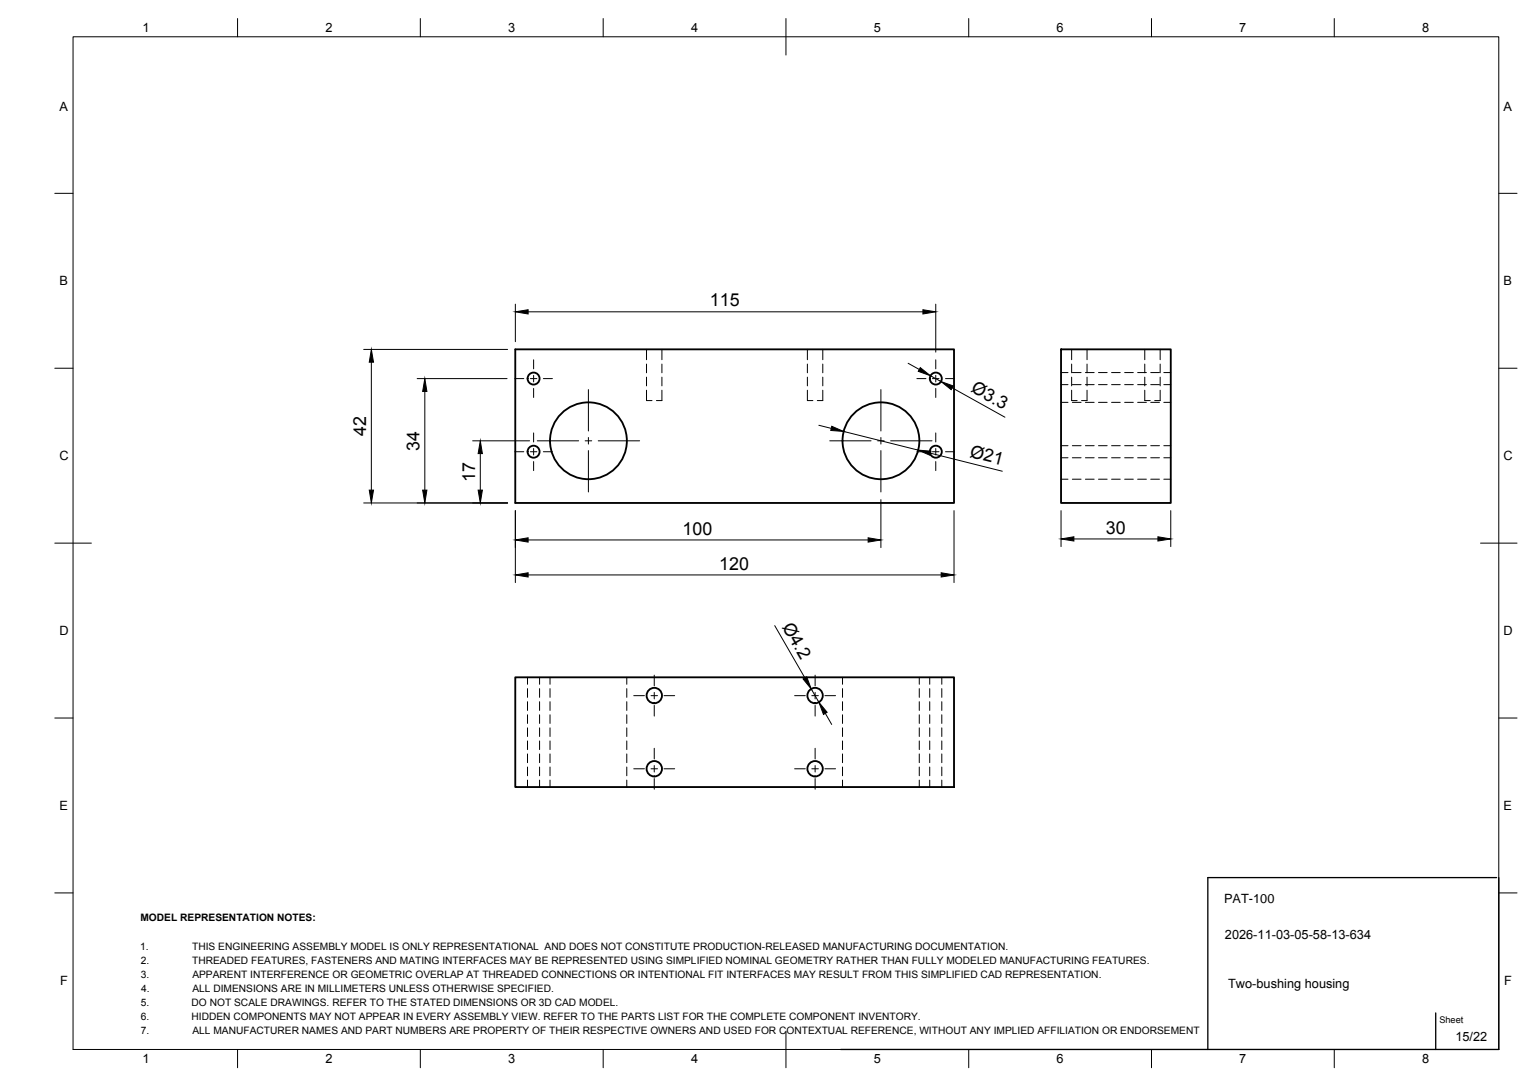
ISO-10303-21;
HEADER;
/* Generated by software containing ST-Developer
 * from STEP Tools, Inc. (www.steptools.com) 
 */

FILE_DESCRIPTION(
/* description */ (''),
/* implementation_level */ '2;1');

FILE_NAME(
/* name */ 'Two-bushing housing.step',
/* time_stamp */ '2026-10-29T16:43:51-07:00',
/* author */ (''),
/* organization */ (''),
/* preprocessor_version */ 'ST-DEVELOPER v20.2',
/* originating_system */ 'Autodesk Translation Framework v15.17.0.0',
/* authorisation */ '');

FILE_SCHEMA (('AUTOMOTIVE_DESIGN { 1 0 10303 214 3 1 1 }'));
ENDSEC;

DATA;
#10=MECHANICAL_DESIGN_GEOMETRIC_PRESENTATION_REPRESENTATION('',(#378),#10292);
#332=SHAPE_REPRESENTATION_RELATIONSHIP('SRR','None',#10429,#355);
#355=ADVANCED_BREP_SHAPE_REPRESENTATION('',(#399),#10281);
#378=STYLED_ITEM('',(#10607),#399);
#399=MANIFOLD_SOLID_BREP('Body1',#5022);
#475=FACE_BOUND('',#1244,.T.);
#476=FACE_BOUND('',#1245,.T.);
#477=FACE_BOUND('',#1246,.T.);
#478=FACE_BOUND('',#1247,.T.);
#479=FACE_BOUND('',#1248,.T.);
#480=FACE_BOUND('',#1249,.T.);
#481=FACE_BOUND('',#1252,.T.);
#482=FACE_BOUND('',#1253,.T.);
#483=FACE_BOUND('',#1254,.T.);
#484=FACE_BOUND('',#1255,.T.);
#485=FACE_BOUND('',#1256,.T.);
#486=FACE_BOUND('',#1257,.T.);
#487=FACE_BOUND('',#1259,.T.);
#488=FACE_BOUND('',#1260,.T.);
#489=FACE_BOUND('',#1261,.T.);
#490=FACE_BOUND('',#1262,.T.);
#634=PLANE('',#5584);
#635=PLANE('',#5588);
#636=PLANE('',#5592);
#637=PLANE('',#5596);
#638=PLANE('',#5603);
#639=PLANE('',#5604);
#640=PLANE('',#5605);
#641=PLANE('',#5606);
#642=PLANE('',#5607);
#643=PLANE('',#5608);
#871=FACE_OUTER_BOUND('',#1228,.T.);
#872=FACE_OUTER_BOUND('',#1229,.T.);
#873=FACE_OUTER_BOUND('',#1230,.T.);
#874=FACE_OUTER_BOUND('',#1231,.T.);
#875=FACE_OUTER_BOUND('',#1232,.T.);
#876=FACE_OUTER_BOUND('',#1233,.T.);
#877=FACE_OUTER_BOUND('',#1234,.T.);
#878=FACE_OUTER_BOUND('',#1235,.T.);
#879=FACE_OUTER_BOUND('',#1236,.T.);
#880=FACE_OUTER_BOUND('',#1237,.T.);
#881=FACE_OUTER_BOUND('',#1238,.T.);
#882=FACE_OUTER_BOUND('',#1239,.T.);
#883=FACE_OUTER_BOUND('',#1240,.T.);
#884=FACE_OUTER_BOUND('',#1241,.T.);
#885=FACE_OUTER_BOUND('',#1242,.T.);
#886=FACE_OUTER_BOUND('',#1243,.T.);
#887=FACE_OUTER_BOUND('',#1250,.T.);
#888=FACE_OUTER_BOUND('',#1251,.T.);
#889=FACE_OUTER_BOUND('',#1258,.T.);
#890=FACE_OUTER_BOUND('',#1263,.T.);
#1228=EDGE_LOOP('',(#4127,#4128,#4129,#4130));
#1229=EDGE_LOOP('',(#4131,#4132,#4133,#4134));
#1230=EDGE_LOOP('',(#4135,#4136,#4137,#4138));
#1231=EDGE_LOOP('',(#4139,#4140,#4141,#4142));
#1232=EDGE_LOOP('',(#4143,#4144,#4145,#4146));
#1233=EDGE_LOOP('',(#4147));
#1234=EDGE_LOOP('',(#4148,#4149,#4150,#4151));
#1235=EDGE_LOOP('',(#4152));
#1236=EDGE_LOOP('',(#4153,#4154,#4155,#4156));
#1237=EDGE_LOOP('',(#4157));
#1238=EDGE_LOOP('',(#4158,#4159,#4160,#4161));
#1239=EDGE_LOOP('',(#4162));
#1240=EDGE_LOOP('',(#4163,#4164,#4165,#4166));
#1241=EDGE_LOOP('',(#4167,#4168,#4169,#4170));
#1242=EDGE_LOOP('',(#4171,#4172,#4173,#4174));
#1243=EDGE_LOOP('',(#4175,#4176,#4177,#4178));
#1244=EDGE_LOOP('',(#4179));
#1245=EDGE_LOOP('',(#4180));
#1246=EDGE_LOOP('',(#4181));
#1247=EDGE_LOOP('',(#4182));
#1248=EDGE_LOOP('',(#4183));
#1249=EDGE_LOOP('',(#4184));
#1250=EDGE_LOOP('',(#4185,#4186,#4187,#4188));
#1251=EDGE_LOOP('',(#4189,#4190,#4191,#4192));
#1252=EDGE_LOOP('',(#4193));
#1253=EDGE_LOOP('',(#4194));
#1254=EDGE_LOOP('',(#4195));
#1255=EDGE_LOOP('',(#4196));
#1256=EDGE_LOOP('',(#4197));
#1257=EDGE_LOOP('',(#4198));
#1258=EDGE_LOOP('',(#4199,#4200,#4201,#4202));
#1259=EDGE_LOOP('',(#4203));
#1260=EDGE_LOOP('',(#4204));
#1261=EDGE_LOOP('',(#4205));
#1262=EDGE_LOOP('',(#4206));
#1263=EDGE_LOOP('',(#4207,#4208,#4209,#4210));
#1644=LINE('',#9621,#2036);
#1645=LINE('',#9627,#2037);
#1646=LINE('',#9633,#2038);
#1647=LINE('',#9639,#2039);
#1648=LINE('',#9645,#2040);
#1649=LINE('',#9652,#2041);
#1650=LINE('',#9659,#2042);
#1651=LINE('',#9666,#2043);
#1652=LINE('',#9673,#2044);
#1653=LINE('',#9679,#2045);
#1654=LINE('',#9684,#2046);
#1655=LINE('',#9686,#2047);
#1656=LINE('',#9688,#2048);
#1657=LINE('',#9689,#2049);
#1658=LINE('',#9692,#2050);
#1659=LINE('',#9694,#2051);
#1660=LINE('',#9695,#2052);
#1661=LINE('',#9698,#2053);
#1662=LINE('',#9700,#2054);
#1663=LINE('',#9701,#2055);
#1664=LINE('',#9703,#2056);
#1665=LINE('',#9704,#2057);
#2036=VECTOR('',#6661,0.165);
#2037=VECTOR('',#6668,0.165);
#2038=VECTOR('',#6675,0.165);
#2039=VECTOR('',#6682,0.165);
#2040=VECTOR('',#6689,0.210000000000001);
#2041=VECTOR('',#6698,0.210000000000001);
#2042=VECTOR('',#6707,0.210000000000001);
#2043=VECTOR('',#6716,0.210000000000001);
#2044=VECTOR('',#6725,1.05);
#2045=VECTOR('',#6732,1.05);
#2046=VECTOR('',#6737,1.);
#2047=VECTOR('',#6738,1.);
#2048=VECTOR('',#6739,1.);
#2049=VECTOR('',#6740,1.);
#2050=VECTOR('',#6743,1.);
#2051=VECTOR('',#6744,1.);
#2052=VECTOR('',#6745,1.);
#2053=VECTOR('',#6748,1.);
#2054=VECTOR('',#6749,1.);
#2055=VECTOR('',#6750,1.);
#2056=VECTOR('',#6753,1.);
#2057=VECTOR('',#6754,1.);
#2298=CIRCLE('',#5570,0.165);
#2299=CIRCLE('',#5571,0.165);
#2300=CIRCLE('',#5573,0.165);
#2301=CIRCLE('',#5574,0.165);
#2302=CIRCLE('',#5576,0.165);
#2303=CIRCLE('',#5577,0.165);
#2304=CIRCLE('',#5579,0.165);
#2305=CIRCLE('',#5580,0.165);
#2306=CIRCLE('',#5582,0.210000000000001);
#2307=CIRCLE('',#5583,0.210000000000001);
#2308=CIRCLE('',#5586,0.210000000000001);
#2309=CIRCLE('',#5587,0.210000000000001);
#2310=CIRCLE('',#5590,0.210000000000001);
#2311=CIRCLE('',#5591,0.210000000000001);
#2312=CIRCLE('',#5594,0.210000000000001);
#2313=CIRCLE('',#5595,0.210000000000001);
#2314=CIRCLE('',#5598,1.05);
#2315=CIRCLE('',#5599,1.05);
#2316=CIRCLE('',#5601,1.05);
#2317=CIRCLE('',#5602,1.05);
#2629=VERTEX_POINT('',#9618);
#2630=VERTEX_POINT('',#9620);
#2631=VERTEX_POINT('',#9624);
#2632=VERTEX_POINT('',#9626);
#2633=VERTEX_POINT('',#9630);
#2634=VERTEX_POINT('',#9632);
#2635=VERTEX_POINT('',#9636);
#2636=VERTEX_POINT('',#9638);
#2637=VERTEX_POINT('',#9642);
#2638=VERTEX_POINT('',#9644);
#2639=VERTEX_POINT('',#9649);
#2640=VERTEX_POINT('',#9651);
#2641=VERTEX_POINT('',#9656);
#2642=VERTEX_POINT('',#9658);
#2643=VERTEX_POINT('',#9663);
#2644=VERTEX_POINT('',#9665);
#2645=VERTEX_POINT('',#9670);
#2646=VERTEX_POINT('',#9672);
#2647=VERTEX_POINT('',#9676);
#2648=VERTEX_POINT('',#9678);
#2649=VERTEX_POINT('',#9682);
#2650=VERTEX_POINT('',#9683);
#2651=VERTEX_POINT('',#9685);
#2652=VERTEX_POINT('',#9687);
#2653=VERTEX_POINT('',#9691);
#2654=VERTEX_POINT('',#9693);
#2655=VERTEX_POINT('',#9697);
#2656=VERTEX_POINT('',#9699);
#3154=EDGE_CURVE('',#2629,#2629,#2298,.T.);
#3155=EDGE_CURVE('',#2629,#2630,#1644,.T.);
#3156=EDGE_CURVE('',#2630,#2630,#2299,.T.);
#3157=EDGE_CURVE('',#2631,#2631,#2300,.T.);
#3158=EDGE_CURVE('',#2631,#2632,#1645,.T.);
#3159=EDGE_CURVE('',#2632,#2632,#2301,.T.);
#3160=EDGE_CURVE('',#2633,#2633,#2302,.T.);
#3161=EDGE_CURVE('',#2633,#2634,#1646,.T.);
#3162=EDGE_CURVE('',#2634,#2634,#2303,.T.);
#3163=EDGE_CURVE('',#2635,#2635,#2304,.T.);
#3164=EDGE_CURVE('',#2635,#2636,#1647,.T.);
#3165=EDGE_CURVE('',#2636,#2636,#2305,.T.);
#3166=EDGE_CURVE('',#2637,#2637,#2306,.T.);
#3167=EDGE_CURVE('',#2637,#2638,#1648,.T.);
#3168=EDGE_CURVE('',#2638,#2638,#2307,.T.);
#3169=EDGE_CURVE('',#2639,#2639,#2308,.T.);
#3170=EDGE_CURVE('',#2639,#2640,#1649,.T.);
#3171=EDGE_CURVE('',#2640,#2640,#2309,.T.);
#3172=EDGE_CURVE('',#2641,#2641,#2310,.T.);
#3173=EDGE_CURVE('',#2641,#2642,#1650,.T.);
#3174=EDGE_CURVE('',#2642,#2642,#2311,.T.);
#3175=EDGE_CURVE('',#2643,#2643,#2312,.T.);
#3176=EDGE_CURVE('',#2643,#2644,#1651,.T.);
#3177=EDGE_CURVE('',#2644,#2644,#2313,.T.);
#3178=EDGE_CURVE('',#2645,#2645,#2314,.T.);
#3179=EDGE_CURVE('',#2645,#2646,#1652,.T.);
#3180=EDGE_CURVE('',#2646,#2646,#2315,.T.);
#3181=EDGE_CURVE('',#2647,#2647,#2316,.T.);
#3182=EDGE_CURVE('',#2647,#2648,#1653,.T.);
#3183=EDGE_CURVE('',#2648,#2648,#2317,.T.);
#3184=EDGE_CURVE('',#2649,#2650,#1654,.T.);
#3185=EDGE_CURVE('',#2650,#2651,#1655,.T.);
#3186=EDGE_CURVE('',#2652,#2651,#1656,.T.);
#3187=EDGE_CURVE('',#2649,#2652,#1657,.T.);
#3188=EDGE_CURVE('',#2653,#2649,#1658,.T.);
#3189=EDGE_CURVE('',#2654,#2652,#1659,.T.);
#3190=EDGE_CURVE('',#2653,#2654,#1660,.T.);
#3191=EDGE_CURVE('',#2655,#2653,#1661,.T.);
#3192=EDGE_CURVE('',#2656,#2654,#1662,.T.);
#3193=EDGE_CURVE('',#2655,#2656,#1663,.T.);
#3194=EDGE_CURVE('',#2650,#2655,#1664,.T.);
#3195=EDGE_CURVE('',#2651,#2656,#1665,.T.);
#4127=ORIENTED_EDGE('',*,*,#3154,.F.);
#4128=ORIENTED_EDGE('',*,*,#3155,.T.);
#4129=ORIENTED_EDGE('',*,*,#3156,.F.);
#4130=ORIENTED_EDGE('',*,*,#3155,.F.);
#4131=ORIENTED_EDGE('',*,*,#3157,.F.);
#4132=ORIENTED_EDGE('',*,*,#3158,.T.);
#4133=ORIENTED_EDGE('',*,*,#3159,.F.);
#4134=ORIENTED_EDGE('',*,*,#3158,.F.);
#4135=ORIENTED_EDGE('',*,*,#3160,.F.);
#4136=ORIENTED_EDGE('',*,*,#3161,.T.);
#4137=ORIENTED_EDGE('',*,*,#3162,.F.);
#4138=ORIENTED_EDGE('',*,*,#3161,.F.);
#4139=ORIENTED_EDGE('',*,*,#3163,.F.);
#4140=ORIENTED_EDGE('',*,*,#3164,.T.);
#4141=ORIENTED_EDGE('',*,*,#3165,.F.);
#4142=ORIENTED_EDGE('',*,*,#3164,.F.);
#4143=ORIENTED_EDGE('',*,*,#3166,.F.);
#4144=ORIENTED_EDGE('',*,*,#3167,.T.);
#4145=ORIENTED_EDGE('',*,*,#3168,.F.);
#4146=ORIENTED_EDGE('',*,*,#3167,.F.);
#4147=ORIENTED_EDGE('',*,*,#3166,.T.);
#4148=ORIENTED_EDGE('',*,*,#3169,.F.);
#4149=ORIENTED_EDGE('',*,*,#3170,.T.);
#4150=ORIENTED_EDGE('',*,*,#3171,.F.);
#4151=ORIENTED_EDGE('',*,*,#3170,.F.);
#4152=ORIENTED_EDGE('',*,*,#3169,.T.);
#4153=ORIENTED_EDGE('',*,*,#3172,.F.);
#4154=ORIENTED_EDGE('',*,*,#3173,.T.);
#4155=ORIENTED_EDGE('',*,*,#3174,.F.);
#4156=ORIENTED_EDGE('',*,*,#3173,.F.);
#4157=ORIENTED_EDGE('',*,*,#3172,.T.);
#4158=ORIENTED_EDGE('',*,*,#3175,.F.);
#4159=ORIENTED_EDGE('',*,*,#3176,.T.);
#4160=ORIENTED_EDGE('',*,*,#3177,.F.);
#4161=ORIENTED_EDGE('',*,*,#3176,.F.);
#4162=ORIENTED_EDGE('',*,*,#3175,.T.);
#4163=ORIENTED_EDGE('',*,*,#3178,.F.);
#4164=ORIENTED_EDGE('',*,*,#3179,.T.);
#4165=ORIENTED_EDGE('',*,*,#3180,.F.);
#4166=ORIENTED_EDGE('',*,*,#3179,.F.);
#4167=ORIENTED_EDGE('',*,*,#3181,.F.);
#4168=ORIENTED_EDGE('',*,*,#3182,.T.);
#4169=ORIENTED_EDGE('',*,*,#3183,.F.);
#4170=ORIENTED_EDGE('',*,*,#3182,.F.);
#4171=ORIENTED_EDGE('',*,*,#3184,.T.);
#4172=ORIENTED_EDGE('',*,*,#3185,.T.);
#4173=ORIENTED_EDGE('',*,*,#3186,.F.);
#4174=ORIENTED_EDGE('',*,*,#3187,.F.);
#4175=ORIENTED_EDGE('',*,*,#3188,.T.);
#4176=ORIENTED_EDGE('',*,*,#3187,.T.);
#4177=ORIENTED_EDGE('',*,*,#3189,.F.);
#4178=ORIENTED_EDGE('',*,*,#3190,.F.);
#4179=ORIENTED_EDGE('',*,*,#3183,.T.);
#4180=ORIENTED_EDGE('',*,*,#3180,.T.);
#4181=ORIENTED_EDGE('',*,*,#3165,.T.);
#4182=ORIENTED_EDGE('',*,*,#3162,.T.);
#4183=ORIENTED_EDGE('',*,*,#3159,.T.);
#4184=ORIENTED_EDGE('',*,*,#3156,.T.);
#4185=ORIENTED_EDGE('',*,*,#3191,.T.);
#4186=ORIENTED_EDGE('',*,*,#3190,.T.);
#4187=ORIENTED_EDGE('',*,*,#3192,.F.);
#4188=ORIENTED_EDGE('',*,*,#3193,.F.);
#4189=ORIENTED_EDGE('',*,*,#3194,.T.);
#4190=ORIENTED_EDGE('',*,*,#3193,.T.);
#4191=ORIENTED_EDGE('',*,*,#3195,.F.);
#4192=ORIENTED_EDGE('',*,*,#3185,.F.);
#4193=ORIENTED_EDGE('',*,*,#3181,.T.);
#4194=ORIENTED_EDGE('',*,*,#3178,.T.);
#4195=ORIENTED_EDGE('',*,*,#3163,.T.);
#4196=ORIENTED_EDGE('',*,*,#3160,.T.);
#4197=ORIENTED_EDGE('',*,*,#3157,.T.);
#4198=ORIENTED_EDGE('',*,*,#3154,.T.);
#4199=ORIENTED_EDGE('',*,*,#3195,.T.);
#4200=ORIENTED_EDGE('',*,*,#3192,.T.);
#4201=ORIENTED_EDGE('',*,*,#3189,.T.);
#4202=ORIENTED_EDGE('',*,*,#3186,.T.);
#4203=ORIENTED_EDGE('',*,*,#3168,.T.);
#4204=ORIENTED_EDGE('',*,*,#3171,.T.);
#4205=ORIENTED_EDGE('',*,*,#3174,.T.);
#4206=ORIENTED_EDGE('',*,*,#3177,.T.);
#4207=ORIENTED_EDGE('',*,*,#3194,.F.);
#4208=ORIENTED_EDGE('',*,*,#3184,.F.);
#4209=ORIENTED_EDGE('',*,*,#3188,.F.);
#4210=ORIENTED_EDGE('',*,*,#3191,.F.);
#4680=CYLINDRICAL_SURFACE('',#5569,0.165);
#4681=CYLINDRICAL_SURFACE('',#5572,0.165);
#4682=CYLINDRICAL_SURFACE('',#5575,0.165);
#4683=CYLINDRICAL_SURFACE('',#5578,0.165);
#4684=CYLINDRICAL_SURFACE('',#5581,0.210000000000001);
#4685=CYLINDRICAL_SURFACE('',#5585,0.210000000000001);
#4686=CYLINDRICAL_SURFACE('',#5589,0.210000000000001);
#4687=CYLINDRICAL_SURFACE('',#5593,0.210000000000001);
#4688=CYLINDRICAL_SURFACE('',#5597,1.05);
#4689=CYLINDRICAL_SURFACE('',#5600,1.05);
#4880=ADVANCED_FACE('',(#871),#4680,.F.);
#4881=ADVANCED_FACE('',(#872),#4681,.F.);
#4882=ADVANCED_FACE('',(#873),#4682,.F.);
#4883=ADVANCED_FACE('',(#874),#4683,.F.);
#4884=ADVANCED_FACE('',(#875),#4684,.F.);
#4885=ADVANCED_FACE('',(#876),#634,.T.);
#4886=ADVANCED_FACE('',(#877),#4685,.F.);
#4887=ADVANCED_FACE('',(#878),#635,.T.);
#4888=ADVANCED_FACE('',(#879),#4686,.F.);
#4889=ADVANCED_FACE('',(#880),#636,.T.);
#4890=ADVANCED_FACE('',(#881),#4687,.F.);
#4891=ADVANCED_FACE('',(#882),#637,.T.);
#4892=ADVANCED_FACE('',(#883),#4688,.F.);
#4893=ADVANCED_FACE('',(#884),#4689,.F.);
#4894=ADVANCED_FACE('',(#885),#638,.T.);
#4895=ADVANCED_FACE('',(#886,#475,#476,#477,#478,#479,#480),#639,.T.);
#4896=ADVANCED_FACE('',(#887),#640,.T.);
#4897=ADVANCED_FACE('',(#888,#481,#482,#483,#484,#485,#486),#641,.T.);
#4898=ADVANCED_FACE('',(#889,#487,#488,#489,#490),#642,.T.);
#4899=ADVANCED_FACE('',(#890),#643,.F.);
#5022=CLOSED_SHELL('',(#4880,#4881,#4882,#4883,#4884,#4885,#4886,#4887,
#4888,#4889,#4890,#4891,#4892,#4893,#4894,#4895,#4896,#4897,#4898,#4899));
#5568=AXIS2_PLACEMENT_3D('',#9616,#6655,#6656);
#5569=AXIS2_PLACEMENT_3D('',#9617,#6657,#6658);
#5570=AXIS2_PLACEMENT_3D('',#9619,#6659,#6660);
#5571=AXIS2_PLACEMENT_3D('',#9622,#6662,#6663);
#5572=AXIS2_PLACEMENT_3D('',#9623,#6664,#6665);
#5573=AXIS2_PLACEMENT_3D('',#9625,#6666,#6667);
#5574=AXIS2_PLACEMENT_3D('',#9628,#6669,#6670);
#5575=AXIS2_PLACEMENT_3D('',#9629,#6671,#6672);
#5576=AXIS2_PLACEMENT_3D('',#9631,#6673,#6674);
#5577=AXIS2_PLACEMENT_3D('',#9634,#6676,#6677);
#5578=AXIS2_PLACEMENT_3D('',#9635,#6678,#6679);
#5579=AXIS2_PLACEMENT_3D('',#9637,#6680,#6681);
#5580=AXIS2_PLACEMENT_3D('',#9640,#6683,#6684);
#5581=AXIS2_PLACEMENT_3D('',#9641,#6685,#6686);
#5582=AXIS2_PLACEMENT_3D('',#9643,#6687,#6688);
#5583=AXIS2_PLACEMENT_3D('',#9646,#6690,#6691);
#5584=AXIS2_PLACEMENT_3D('',#9647,#6692,#6693);
#5585=AXIS2_PLACEMENT_3D('',#9648,#6694,#6695);
#5586=AXIS2_PLACEMENT_3D('',#9650,#6696,#6697);
#5587=AXIS2_PLACEMENT_3D('',#9653,#6699,#6700);
#5588=AXIS2_PLACEMENT_3D('',#9654,#6701,#6702);
#5589=AXIS2_PLACEMENT_3D('',#9655,#6703,#6704);
#5590=AXIS2_PLACEMENT_3D('',#9657,#6705,#6706);
#5591=AXIS2_PLACEMENT_3D('',#9660,#6708,#6709);
#5592=AXIS2_PLACEMENT_3D('',#9661,#6710,#6711);
#5593=AXIS2_PLACEMENT_3D('',#9662,#6712,#6713);
#5594=AXIS2_PLACEMENT_3D('',#9664,#6714,#6715);
#5595=AXIS2_PLACEMENT_3D('',#9667,#6717,#6718);
#5596=AXIS2_PLACEMENT_3D('',#9668,#6719,#6720);
#5597=AXIS2_PLACEMENT_3D('',#9669,#6721,#6722);
#5598=AXIS2_PLACEMENT_3D('',#9671,#6723,#6724);
#5599=AXIS2_PLACEMENT_3D('',#9674,#6726,#6727);
#5600=AXIS2_PLACEMENT_3D('',#9675,#6728,#6729);
#5601=AXIS2_PLACEMENT_3D('',#9677,#6730,#6731);
#5602=AXIS2_PLACEMENT_3D('',#9680,#6733,#6734);
#5603=AXIS2_PLACEMENT_3D('',#9681,#6735,#6736);
#5604=AXIS2_PLACEMENT_3D('',#9690,#6741,#6742);
#5605=AXIS2_PLACEMENT_3D('',#9696,#6746,#6747);
#5606=AXIS2_PLACEMENT_3D('',#9702,#6751,#6752);
#5607=AXIS2_PLACEMENT_3D('',#9705,#6755,#6756);
#5608=AXIS2_PLACEMENT_3D('',#9706,#6757,#6758);
#6655=DIRECTION('axis',(0.,0.,1.));
#6656=DIRECTION('refdir',(1.,0.,0.));
#6657=DIRECTION('center_axis',(1.,0.,0.));
#6658=DIRECTION('ref_axis',(0.,0.,-1.));
#6659=DIRECTION('center_axis',(1.,0.,0.));
#6660=DIRECTION('ref_axis',(0.,0.,-1.));
#6661=DIRECTION('',(1.,0.,0.));
#6662=DIRECTION('center_axis',(-1.,0.,0.));
#6663=DIRECTION('ref_axis',(0.,0.,-1.));
#6664=DIRECTION('center_axis',(1.,0.,0.));
#6665=DIRECTION('ref_axis',(0.,0.,-1.));
#6666=DIRECTION('center_axis',(1.,0.,0.));
#6667=DIRECTION('ref_axis',(0.,0.,-1.));
#6668=DIRECTION('',(1.,0.,0.));
#6669=DIRECTION('center_axis',(-1.,0.,0.));
#6670=DIRECTION('ref_axis',(0.,0.,-1.));
#6671=DIRECTION('center_axis',(1.,0.,0.));
#6672=DIRECTION('ref_axis',(0.,0.,-1.));
#6673=DIRECTION('center_axis',(1.,0.,0.));
#6674=DIRECTION('ref_axis',(0.,0.,-1.));
#6675=DIRECTION('',(1.,0.,0.));
#6676=DIRECTION('center_axis',(-1.,0.,0.));
#6677=DIRECTION('ref_axis',(0.,0.,-1.));
#6678=DIRECTION('center_axis',(1.,0.,0.));
#6679=DIRECTION('ref_axis',(0.,0.,-1.));
#6680=DIRECTION('center_axis',(1.,0.,0.));
#6681=DIRECTION('ref_axis',(0.,0.,-1.));
#6682=DIRECTION('',(1.,0.,0.));
#6683=DIRECTION('center_axis',(-1.,0.,0.));
#6684=DIRECTION('ref_axis',(0.,0.,-1.));
#6685=DIRECTION('center_axis',(0.,0.,1.));
#6686=DIRECTION('ref_axis',(1.,0.,0.));
#6687=DIRECTION('center_axis',(0.,0.,1.));
#6688=DIRECTION('ref_axis',(1.,0.,0.));
#6689=DIRECTION('',(0.,0.,1.));
#6690=DIRECTION('center_axis',(0.,0.,-1.));
#6691=DIRECTION('ref_axis',(1.,0.,0.));
#6692=DIRECTION('center_axis',(0.,0.,1.));
#6693=DIRECTION('ref_axis',(1.,0.,0.));
#6694=DIRECTION('center_axis',(0.,0.,1.));
#6695=DIRECTION('ref_axis',(1.,0.,0.));
#6696=DIRECTION('center_axis',(0.,0.,1.));
#6697=DIRECTION('ref_axis',(1.,0.,0.));
#6698=DIRECTION('',(0.,0.,1.));
#6699=DIRECTION('center_axis',(0.,0.,-1.));
#6700=DIRECTION('ref_axis',(1.,0.,0.));
#6701=DIRECTION('center_axis',(0.,0.,1.));
#6702=DIRECTION('ref_axis',(1.,0.,0.));
#6703=DIRECTION('center_axis',(0.,0.,1.));
#6704=DIRECTION('ref_axis',(1.,0.,0.));
#6705=DIRECTION('center_axis',(0.,0.,1.));
#6706=DIRECTION('ref_axis',(1.,0.,0.));
#6707=DIRECTION('',(0.,0.,1.));
#6708=DIRECTION('center_axis',(0.,0.,-1.));
#6709=DIRECTION('ref_axis',(1.,0.,0.));
#6710=DIRECTION('center_axis',(0.,0.,1.));
#6711=DIRECTION('ref_axis',(1.,0.,0.));
#6712=DIRECTION('center_axis',(0.,0.,1.));
#6713=DIRECTION('ref_axis',(1.,0.,0.));
#6714=DIRECTION('center_axis',(0.,0.,1.));
#6715=DIRECTION('ref_axis',(1.,0.,0.));
#6716=DIRECTION('',(0.,0.,1.));
#6717=DIRECTION('center_axis',(0.,0.,-1.));
#6718=DIRECTION('ref_axis',(1.,0.,0.));
#6719=DIRECTION('center_axis',(0.,0.,1.));
#6720=DIRECTION('ref_axis',(1.,0.,0.));
#6721=DIRECTION('center_axis',(1.,0.,0.));
#6722=DIRECTION('ref_axis',(0.,0.,-1.));
#6723=DIRECTION('center_axis',(1.,0.,0.));
#6724=DIRECTION('ref_axis',(0.,0.,-1.));
#6725=DIRECTION('',(1.,0.,0.));
#6726=DIRECTION('center_axis',(-1.,0.,0.));
#6727=DIRECTION('ref_axis',(0.,0.,-1.));
#6728=DIRECTION('center_axis',(1.,0.,0.));
#6729=DIRECTION('ref_axis',(0.,0.,-1.));
#6730=DIRECTION('center_axis',(1.,0.,0.));
#6731=DIRECTION('ref_axis',(0.,0.,-1.));
#6732=DIRECTION('',(1.,0.,0.));
#6733=DIRECTION('center_axis',(-1.,0.,0.));
#6734=DIRECTION('ref_axis',(0.,0.,-1.));
#6735=DIRECTION('center_axis',(0.,1.,0.));
#6736=DIRECTION('ref_axis',(-1.,0.,0.));
#6737=DIRECTION('',(-1.,0.,0.));
#6738=DIRECTION('',(0.,0.,1.));
#6739=DIRECTION('',(-1.,0.,0.));
#6740=DIRECTION('',(0.,0.,1.));
#6741=DIRECTION('center_axis',(1.,0.,0.));
#6742=DIRECTION('ref_axis',(0.,1.,0.));
#6743=DIRECTION('',(0.,1.,0.));
#6744=DIRECTION('',(0.,1.,0.));
#6745=DIRECTION('',(0.,0.,1.));
#6746=DIRECTION('center_axis',(0.,-1.,0.));
#6747=DIRECTION('ref_axis',(1.,0.,0.));
#6748=DIRECTION('',(1.,0.,0.));
#6749=DIRECTION('',(1.,0.,0.));
#6750=DIRECTION('',(0.,0.,1.));
#6751=DIRECTION('center_axis',(-1.,0.,0.));
#6752=DIRECTION('ref_axis',(0.,-1.,0.));
#6753=DIRECTION('',(0.,-1.,0.));
#6754=DIRECTION('',(0.,-1.,0.));
#6755=DIRECTION('center_axis',(0.,0.,1.));
#6756=DIRECTION('ref_axis',(1.,0.,0.));
#6757=DIRECTION('center_axis',(0.,0.,1.));
#6758=DIRECTION('ref_axis',(1.,0.,0.));
#9616=CARTESIAN_POINT('',(0.,0.,0.));
#9617=CARTESIAN_POINT('Origin',(13.4,5.5,3.));
#9618=CARTESIAN_POINT('',(13.5,5.5,3.165));
#9619=CARTESIAN_POINT('Origin',(13.5,5.5,3.));
#9620=CARTESIAN_POINT('',(16.5,5.5,3.165));
#9621=CARTESIAN_POINT('',(13.4,5.5,3.165));
#9622=CARTESIAN_POINT('Origin',(16.5,5.5,3.));
#9623=CARTESIAN_POINT('Origin',(13.4,-5.5,5.));
#9624=CARTESIAN_POINT('',(13.5,-5.5,5.165));
#9625=CARTESIAN_POINT('Origin',(13.5,-5.5,5.));
#9626=CARTESIAN_POINT('',(16.5,-5.5,5.165));
#9627=CARTESIAN_POINT('',(13.4,-5.5,5.165));
#9628=CARTESIAN_POINT('Origin',(16.5,-5.5,5.));
#9629=CARTESIAN_POINT('Origin',(13.4,-5.5,3.));
#9630=CARTESIAN_POINT('',(13.5,-5.5,3.165));
#9631=CARTESIAN_POINT('Origin',(13.5,-5.5,3.));
#9632=CARTESIAN_POINT('',(16.5,-5.5,3.165));
#9633=CARTESIAN_POINT('',(13.4,-5.5,3.165));
#9634=CARTESIAN_POINT('Origin',(16.5,-5.5,3.));
#9635=CARTESIAN_POINT('Origin',(13.4,5.5,5.));
#9636=CARTESIAN_POINT('',(13.5,5.5,5.165));
#9637=CARTESIAN_POINT('Origin',(13.5,5.5,5.));
#9638=CARTESIAN_POINT('',(16.5,5.5,5.165));
#9639=CARTESIAN_POINT('',(13.4,5.5,5.165));
#9640=CARTESIAN_POINT('Origin',(16.5,5.5,5.));
#9641=CARTESIAN_POINT('Origin',(16.,-2.2,4.4));
#9642=CARTESIAN_POINT('',(15.79,-2.2,4.4));
#9643=CARTESIAN_POINT('Origin',(16.,-2.2,4.4));
#9644=CARTESIAN_POINT('',(15.79,-2.2,5.8));
#9645=CARTESIAN_POINT('',(15.79,-2.2,4.4));
#9646=CARTESIAN_POINT('Origin',(16.,-2.2,5.8));
#9647=CARTESIAN_POINT('Origin',(16.,-2.2,4.4));
#9648=CARTESIAN_POINT('Origin',(14.,2.2,4.4));
#9649=CARTESIAN_POINT('',(13.79,2.2,4.4));
#9650=CARTESIAN_POINT('Origin',(14.,2.2,4.4));
#9651=CARTESIAN_POINT('',(13.79,2.2,5.8));
#9652=CARTESIAN_POINT('',(13.79,2.2,4.4));
#9653=CARTESIAN_POINT('Origin',(14.,2.2,5.8));
#9654=CARTESIAN_POINT('Origin',(14.,2.2,4.4));
#9655=CARTESIAN_POINT('Origin',(14.,-2.2,4.4));
#9656=CARTESIAN_POINT('',(13.79,-2.2,4.4));
#9657=CARTESIAN_POINT('Origin',(14.,-2.2,4.4));
#9658=CARTESIAN_POINT('',(13.79,-2.2,5.8));
#9659=CARTESIAN_POINT('',(13.79,-2.2,4.4));
#9660=CARTESIAN_POINT('Origin',(14.,-2.2,5.8));
#9661=CARTESIAN_POINT('Origin',(14.,-2.2,4.4));
#9662=CARTESIAN_POINT('Origin',(16.,2.2,4.4));
#9663=CARTESIAN_POINT('',(15.79,2.2,4.4));
#9664=CARTESIAN_POINT('Origin',(16.,2.2,4.4));
#9665=CARTESIAN_POINT('',(15.79,2.2,5.8));
#9666=CARTESIAN_POINT('',(15.79,2.2,4.4));
#9667=CARTESIAN_POINT('Origin',(16.,2.2,5.8));
#9668=CARTESIAN_POINT('Origin',(16.,2.2,4.4));
#9669=CARTESIAN_POINT('Origin',(13.4,-4.,3.3));
#9670=CARTESIAN_POINT('',(13.5,-4.,4.35));
#9671=CARTESIAN_POINT('Origin',(13.5,-4.,3.3));
#9672=CARTESIAN_POINT('',(16.5,-4.,4.35));
#9673=CARTESIAN_POINT('',(13.4,-4.,4.35));
#9674=CARTESIAN_POINT('Origin',(16.5,-4.,3.3));
#9675=CARTESIAN_POINT('Origin',(13.4,4.,3.3));
#9676=CARTESIAN_POINT('',(13.5,4.,4.35));
#9677=CARTESIAN_POINT('Origin',(13.5,4.,3.3));
#9678=CARTESIAN_POINT('',(16.5,4.,4.35));
#9679=CARTESIAN_POINT('',(13.4,4.,4.35));
#9680=CARTESIAN_POINT('Origin',(16.5,4.,3.3));
#9681=CARTESIAN_POINT('Origin',(16.5,6.,1.6));
#9682=CARTESIAN_POINT('',(16.5,6.,1.6));
#9683=CARTESIAN_POINT('',(13.5,6.,1.6));
#9684=CARTESIAN_POINT('',(16.5,6.,1.6));
#9685=CARTESIAN_POINT('',(13.5,6.,5.8));
#9686=CARTESIAN_POINT('',(13.5,6.,1.6));
#9687=CARTESIAN_POINT('',(16.5,6.,5.8));
#9688=CARTESIAN_POINT('',(16.5,6.,5.8));
#9689=CARTESIAN_POINT('',(16.5,6.,1.6));
#9690=CARTESIAN_POINT('Origin',(16.5,-6.,1.6));
#9691=CARTESIAN_POINT('',(16.5,-6.,1.6));
#9692=CARTESIAN_POINT('',(16.5,-6.,1.6));
#9693=CARTESIAN_POINT('',(16.5,-6.,5.8));
#9694=CARTESIAN_POINT('',(16.5,-6.,5.8));
#9695=CARTESIAN_POINT('',(16.5,-6.,1.6));
#9696=CARTESIAN_POINT('Origin',(13.5,-6.,1.6));
#9697=CARTESIAN_POINT('',(13.5,-6.,1.6));
#9698=CARTESIAN_POINT('',(13.5,-6.,1.6));
#9699=CARTESIAN_POINT('',(13.5,-6.,5.8));
#9700=CARTESIAN_POINT('',(13.5,-6.,5.8));
#9701=CARTESIAN_POINT('',(13.5,-6.,1.6));
#9702=CARTESIAN_POINT('Origin',(13.5,6.,1.6));
#9703=CARTESIAN_POINT('',(13.5,6.,1.6));
#9704=CARTESIAN_POINT('',(13.5,6.,5.8));
#9705=CARTESIAN_POINT('Origin',(15.,0.,5.8));
#9706=CARTESIAN_POINT('Origin',(15.,0.,1.6));
#10253=UNCERTAINTY_MEASURE_WITH_UNIT(LENGTH_MEASURE(0.001),#10293,
'DISTANCE_ACCURACY_VALUE',
'Maximum model space distance between geometric entities at asserted c
onnectivities');
#10264=UNCERTAINTY_MEASURE_WITH_UNIT(LENGTH_MEASURE(0.001),#10293,
'DISTANCE_ACCURACY_VALUE',
'Maximum model space distance between geometric entities at asserted c
onnectivities');
#10281=(
GEOMETRIC_REPRESENTATION_CONTEXT(3)
GLOBAL_UNCERTAINTY_ASSIGNED_CONTEXT((#10253))
GLOBAL_UNIT_ASSIGNED_CONTEXT((#10293,#10295,#10296))
REPRESENTATION_CONTEXT('','3D')
);
#10292=(
GEOMETRIC_REPRESENTATION_CONTEXT(3)
GLOBAL_UNCERTAINTY_ASSIGNED_CONTEXT((#10264))
GLOBAL_UNIT_ASSIGNED_CONTEXT((#10293,#10295,#10296))
REPRESENTATION_CONTEXT('','3D')
);
#10293=(
LENGTH_UNIT()
NAMED_UNIT(*)
SI_UNIT(.CENTI.,.METRE.)
);
#10295=(
NAMED_UNIT(*)
PLANE_ANGLE_UNIT()
SI_UNIT($,.RADIAN.)
);
#10296=(
NAMED_UNIT(*)
SI_UNIT($,.STERADIAN.)
SOLID_ANGLE_UNIT()
);
#10313=SHAPE_DEFINITION_REPRESENTATION(#10340,#10429);
#10340=PRODUCT_DEFINITION_SHAPE('',$,#10457);
#10429=SHAPE_REPRESENTATION('',(#5568),#10281);
#10440=PRODUCT_DEFINITION_CONTEXT('part definition',#10523,'design');
#10457=PRODUCT_DEFINITION('Two-bushing housing',
'Two-bushing housing',#10484,#10440);
#10484=PRODUCT_DEFINITION_FORMATION('',$,#10541);
#10523=APPLICATION_CONTEXT(
'Core Data for Automotive Mechanical Design Process');
#10524=PRODUCT_CONTEXT('part definition',#10523,'mechanical');
#10541=PRODUCT('Two-bushing housing','Two-bushing housing',
'Two-bushing housing',(#10524));
#10601=COLOUR_RGB('Dark Blue',0.08,0.2,0.34);
#10602=FILL_AREA_STYLE_COLOUR('',#10601);
#10603=FILL_AREA_STYLE('',(#10602));
#10604=SURFACE_STYLE_FILL_AREA(#10603);
#10605=SURFACE_SIDE_STYLE('',(#10604));
#10606=SURFACE_STYLE_USAGE(.BOTH.,#10605);
#10607=PRESENTATION_STYLE_ASSIGNMENT((#10606));
ENDSEC;
END-ISO-10303-21;
